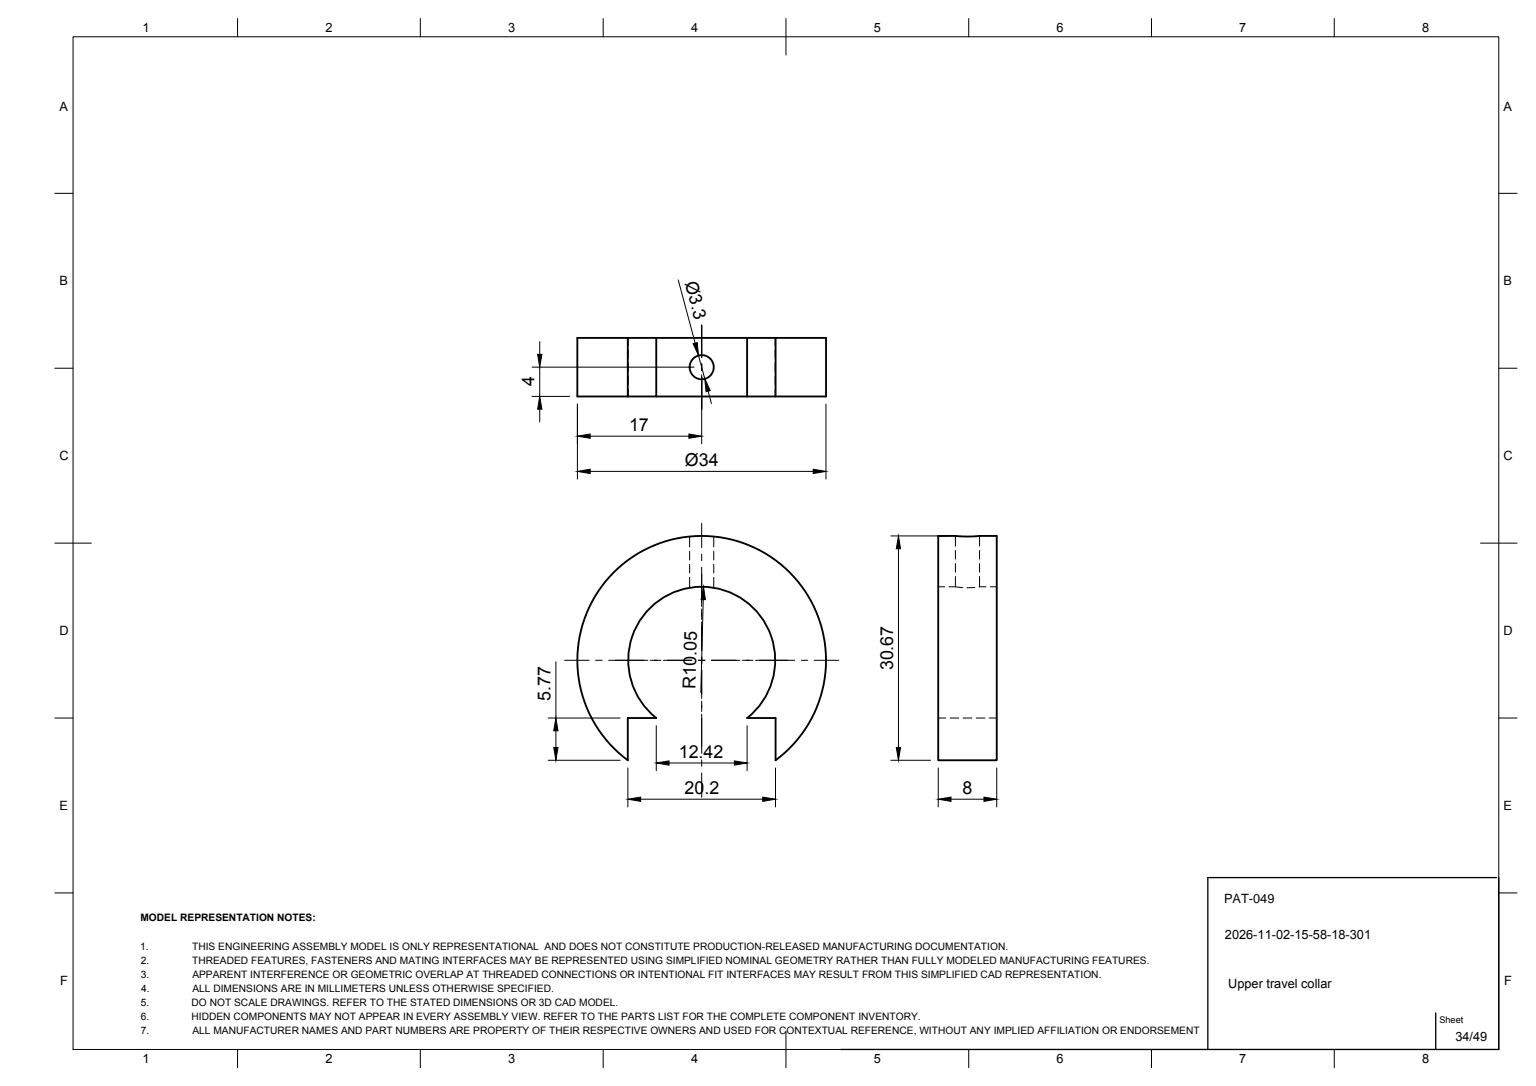
ISO-10303-21;
HEADER;
/* Generated by software containing ST-Developer
 * from STEP Tools, Inc. (www.steptools.com) 
 */

FILE_DESCRIPTION(
/* description */ ('Hand drill press frame (manual)'),
/* implementation_level */ '2;1');

FILE_NAME(
/* name */ 'Upper travel collar.step',
/* time_stamp */ '2026-10-28T03:25:28-07:00',
/* author */ (''),
/* organization */ (''),
/* preprocessor_version */ 'ST-DEVELOPER v20.2',
/* originating_system */ 'Autodesk Translation Framework v15.17.0.0',
/* authorisation */ '');

FILE_SCHEMA (('AUTOMOTIVE_DESIGN { 1 0 10303 214 3 1 1 }'));
ENDSEC;

DATA;
#10=MECHANICAL_DESIGN_GEOMETRIC_PRESENTATION_REPRESENTATION('',(#653),#33299);
#525=B_SPLINE_CURVE_WITH_KNOTS('',3,(#20892,#20893,#20894,#20895,#20896,
#20897,#20898,#20899,#20900,#20901),.UNSPECIFIED.,.F.,.F.,(4,2,2,2,4),(0.,
0.062275384959466,0.124550769918932,0.186824589898798,0.249098409878663),
 .UNSPECIFIED.);
#526=B_SPLINE_CURVE_WITH_KNOTS('',3,(#20902,#20903,#20904,#20905,#20906,
#20907,#20908,#20909,#20910,#20911,#20912,#20913,#20914,#20915,#20916,#20917,
#20918,#20919,#20920,#20921,#20922,#20923,#20924,#20925,#20926,#20927),
 .UNSPECIFIED.,.F.,.F.,(4,2,2,2,2,2,2,2,2,2,2,2,4),(0.249098409878663,0.311372229858529,
0.373646049838394,0.43592143479786,0.498196819757326,0.560472204716792,
0.622747589676259,0.685021409656124,0.74729522963599,0.809569049615855,
0.871842869595721,0.934118254555187,0.996393639514653),.UNSPECIFIED.);
#527=B_SPLINE_CURVE_WITH_KNOTS('',3,(#20931,#20932,#20933,#20934,#20935,
#20936,#20937,#20938,#20939,#20940,#20941,#20942,#20943,#20944,#20945,#20946,
#20947,#20948,#20949,#20950,#20951,#20952,#20953,#20954,#20955,#20956),
 .UNSPECIFIED.,.F.,.F.,(4,2,2,2,2,2,2,2,2,2,2,2,4),(0.,0.0621954302022363,
0.124390860404473,0.186586102839084,0.248781345273696,0.310976587708308,
0.37317183014292,0.435367260345156,0.497562690547392,0.559758120749629,
0.621953550951865,0.684148793386477,0.746344035821089),.UNSPECIFIED.);
#528=B_SPLINE_CURVE_WITH_KNOTS('',3,(#20957,#20958,#20959,#20960,#20961,
#20962,#20963,#20964,#20965,#20966),.UNSPECIFIED.,.F.,.F.,(4,2,2,2,4),(0.746344035821089,
0.8085392782557,0.870734520690312,0.932929950892549,0.995125381094785),
 .UNSPECIFIED.);
#556=SHAPE_REPRESENTATION_RELATIONSHIP('SRR','None',#33517,#601);
#601=ADVANCED_BREP_SHAPE_REPRESENTATION('',(#704),#33279);
#653=STYLED_ITEM('',(#33800),#704);
#704=MANIFOLD_SOLID_BREP('Body1',#12672);
#852=FACE_BOUND('',#2635,.T.);
#853=FACE_BOUND('',#2637,.T.);
#1223=PLANE('',#13969);
#1224=PLANE('',#13970);
#1225=PLANE('',#13971);
#1226=PLANE('',#13972);
#1227=PLANE('',#13973);
#1228=PLANE('',#13980);
#1807=FACE_OUTER_BOUND('',#2628,.T.);
#1808=FACE_OUTER_BOUND('',#2629,.T.);
#1809=FACE_OUTER_BOUND('',#2630,.T.);
#1810=FACE_OUTER_BOUND('',#2631,.T.);
#1811=FACE_OUTER_BOUND('',#2632,.T.);
#1812=FACE_OUTER_BOUND('',#2633,.T.);
#1813=FACE_OUTER_BOUND('',#2634,.T.);
#1814=FACE_OUTER_BOUND('',#2636,.T.);
#1815=FACE_OUTER_BOUND('',#2638,.T.);
#2628=EDGE_LOOP('',(#10769,#10770,#10771,#10772,#10773,#10774));
#2629=EDGE_LOOP('',(#10775,#10776,#10777,#10778));
#2630=EDGE_LOOP('',(#10779,#10780,#10781,#10782));
#2631=EDGE_LOOP('',(#10783,#10784,#10785,#10786));
#2632=EDGE_LOOP('',(#10787,#10788,#10789,#10790));
#2633=EDGE_LOOP('',(#10791,#10792,#10793,#10794,#10795,#10796));
#2634=EDGE_LOOP('',(#10797,#10798,#10799,#10800));
#2635=EDGE_LOOP('',(#10801,#10802));
#2636=EDGE_LOOP('',(#10803,#10804,#10805,#10806));
#2637=EDGE_LOOP('',(#10807,#10808));
#2638=EDGE_LOOP('',(#10809,#10810,#10811,#10812,#10813,#10814));
#3749=LINE('',#20929,#4914);
#3750=LINE('',#20970,#4915);
#3751=LINE('',#20972,#4916);
#3752=LINE('',#20974,#4917);
#3753=LINE('',#20975,#4918);
#3754=LINE('',#20979,#4919);
#3755=LINE('',#20981,#4920);
#3756=LINE('',#20983,#4921);
#3757=LINE('',#20984,#4922);
#3758=LINE('',#20987,#4923);
#3759=LINE('',#20989,#4924);
#3760=LINE('',#20990,#4925);
#3761=LINE('',#20993,#4926);
#3762=LINE('',#20995,#4927);
#3763=LINE('',#20996,#4928);
#4914=VECTOR('',#16794,0.164999999999999);
#4915=VECTOR('',#16797,1.);
#4916=VECTOR('',#16798,1.);
#4917=VECTOR('',#16799,1.);
#4918=VECTOR('',#16800,1.);
#4919=VECTOR('',#16803,1.);
#4920=VECTOR('',#16804,1.);
#4921=VECTOR('',#16805,1.);
#4922=VECTOR('',#16806,1.);
#4923=VECTOR('',#16809,1.);
#4924=VECTOR('',#16810,1.);
#4925=VECTOR('',#16811,1.);
#4926=VECTOR('',#16814,1.);
#4927=VECTOR('',#16815,1.);
#4928=VECTOR('',#16816,1.);
#5489=CIRCLE('',#13974,1.005);
#5490=CIRCLE('',#13975,1.7);
#5491=CIRCLE('',#13977,1.7);
#5492=CIRCLE('',#13979,1.005);
#6403=VERTEX_POINT('',#20890);
#6404=VERTEX_POINT('',#20891);
#6405=VERTEX_POINT('',#20928);
#6406=VERTEX_POINT('',#20930);
#6407=VERTEX_POINT('',#20968);
#6408=VERTEX_POINT('',#20969);
#6409=VERTEX_POINT('',#20971);
#6410=VERTEX_POINT('',#20973);
#6411=VERTEX_POINT('',#20977);
#6412=VERTEX_POINT('',#20978);
#6413=VERTEX_POINT('',#20980);
#6414=VERTEX_POINT('',#20982);
#6415=VERTEX_POINT('',#20986);
#6416=VERTEX_POINT('',#20988);
#6417=VERTEX_POINT('',#20992);
#6418=VERTEX_POINT('',#20994);
#7913=EDGE_CURVE('',#6403,#6404,#525,.T.);
#7914=EDGE_CURVE('',#6404,#6403,#526,.T.);
#7915=EDGE_CURVE('',#6404,#6405,#3749,.T.);
#7916=EDGE_CURVE('',#6406,#6405,#527,.T.);
#7917=EDGE_CURVE('',#6405,#6406,#528,.T.);
#7918=EDGE_CURVE('',#6407,#6408,#3750,.T.);
#7919=EDGE_CURVE('',#6407,#6409,#3751,.T.);
#7920=EDGE_CURVE('',#6410,#6409,#3752,.T.);
#7921=EDGE_CURVE('',#6408,#6410,#3753,.T.);
#7922=EDGE_CURVE('',#6411,#6412,#3754,.T.);
#7923=EDGE_CURVE('',#6411,#6413,#3755,.T.);
#7924=EDGE_CURVE('',#6414,#6413,#3756,.T.);
#7925=EDGE_CURVE('',#6412,#6414,#3757,.T.);
#7926=EDGE_CURVE('',#6415,#6407,#3758,.T.);
#7927=EDGE_CURVE('',#6416,#6415,#3759,.T.);
#7928=EDGE_CURVE('',#6409,#6416,#3760,.T.);
#7929=EDGE_CURVE('',#6417,#6411,#3761,.T.);
#7930=EDGE_CURVE('',#6418,#6417,#3762,.T.);
#7931=EDGE_CURVE('',#6413,#6418,#3763,.T.);
#7932=EDGE_CURVE('',#6416,#6414,#5489,.T.);
#7933=EDGE_CURVE('',#6418,#6410,#5490,.T.);
#7934=EDGE_CURVE('',#6417,#6408,#5491,.T.);
#7935=EDGE_CURVE('',#6415,#6412,#5492,.T.);
#10769=ORIENTED_EDGE('',*,*,#7913,.F.);
#10770=ORIENTED_EDGE('',*,*,#7914,.F.);
#10771=ORIENTED_EDGE('',*,*,#7915,.T.);
#10772=ORIENTED_EDGE('',*,*,#7916,.F.);
#10773=ORIENTED_EDGE('',*,*,#7917,.F.);
#10774=ORIENTED_EDGE('',*,*,#7915,.F.);
#10775=ORIENTED_EDGE('',*,*,#7918,.F.);
#10776=ORIENTED_EDGE('',*,*,#7919,.T.);
#10777=ORIENTED_EDGE('',*,*,#7920,.F.);
#10778=ORIENTED_EDGE('',*,*,#7921,.F.);
#10779=ORIENTED_EDGE('',*,*,#7922,.F.);
#10780=ORIENTED_EDGE('',*,*,#7923,.T.);
#10781=ORIENTED_EDGE('',*,*,#7924,.F.);
#10782=ORIENTED_EDGE('',*,*,#7925,.F.);
#10783=ORIENTED_EDGE('',*,*,#7926,.F.);
#10784=ORIENTED_EDGE('',*,*,#7927,.F.);
#10785=ORIENTED_EDGE('',*,*,#7928,.F.);
#10786=ORIENTED_EDGE('',*,*,#7919,.F.);
#10787=ORIENTED_EDGE('',*,*,#7929,.F.);
#10788=ORIENTED_EDGE('',*,*,#7930,.F.);
#10789=ORIENTED_EDGE('',*,*,#7931,.F.);
#10790=ORIENTED_EDGE('',*,*,#7923,.F.);
#10791=ORIENTED_EDGE('',*,*,#7920,.T.);
#10792=ORIENTED_EDGE('',*,*,#7928,.T.);
#10793=ORIENTED_EDGE('',*,*,#7932,.T.);
#10794=ORIENTED_EDGE('',*,*,#7924,.T.);
#10795=ORIENTED_EDGE('',*,*,#7931,.T.);
#10796=ORIENTED_EDGE('',*,*,#7933,.T.);
#10797=ORIENTED_EDGE('',*,*,#7921,.T.);
#10798=ORIENTED_EDGE('',*,*,#7933,.F.);
#10799=ORIENTED_EDGE('',*,*,#7930,.T.);
#10800=ORIENTED_EDGE('',*,*,#7934,.T.);
#10801=ORIENTED_EDGE('',*,*,#7916,.T.);
#10802=ORIENTED_EDGE('',*,*,#7917,.T.);
#10803=ORIENTED_EDGE('',*,*,#7927,.T.);
#10804=ORIENTED_EDGE('',*,*,#7935,.T.);
#10805=ORIENTED_EDGE('',*,*,#7925,.T.);
#10806=ORIENTED_EDGE('',*,*,#7932,.F.);
#10807=ORIENTED_EDGE('',*,*,#7913,.T.);
#10808=ORIENTED_EDGE('',*,*,#7914,.T.);
#10809=ORIENTED_EDGE('',*,*,#7918,.T.);
#10810=ORIENTED_EDGE('',*,*,#7934,.F.);
#10811=ORIENTED_EDGE('',*,*,#7929,.T.);
#10812=ORIENTED_EDGE('',*,*,#7922,.T.);
#10813=ORIENTED_EDGE('',*,*,#7935,.F.);
#10814=ORIENTED_EDGE('',*,*,#7926,.T.);
#11893=CYLINDRICAL_SURFACE('',#13968,0.164999999999999);
#11894=CYLINDRICAL_SURFACE('',#13976,1.7);
#11895=CYLINDRICAL_SURFACE('',#13978,1.005);
#12416=ADVANCED_FACE('',(#1807),#11893,.F.);
#12417=ADVANCED_FACE('',(#1808),#1223,.F.);
#12418=ADVANCED_FACE('',(#1809),#1224,.F.);
#12419=ADVANCED_FACE('',(#1810),#1225,.F.);
#12420=ADVANCED_FACE('',(#1811),#1226,.F.);
#12421=ADVANCED_FACE('',(#1812),#1227,.T.);
#12422=ADVANCED_FACE('',(#1813,#852),#11894,.T.);
#12423=ADVANCED_FACE('',(#1814,#853),#11895,.F.);
#12424=ADVANCED_FACE('',(#1815),#1228,.F.);
#12672=CLOSED_SHELL('',(#12416,#12417,#12418,#12419,#12420,#12421,#12422,
#12423,#12424));
#13967=AXIS2_PLACEMENT_3D('',#20888,#16790,#16791);
#13968=AXIS2_PLACEMENT_3D('',#20889,#16792,#16793);
#13969=AXIS2_PLACEMENT_3D('',#20967,#16795,#16796);
#13970=AXIS2_PLACEMENT_3D('',#20976,#16801,#16802);
#13971=AXIS2_PLACEMENT_3D('',#20985,#16807,#16808);
#13972=AXIS2_PLACEMENT_3D('',#20991,#16812,#16813);
#13973=AXIS2_PLACEMENT_3D('',#20997,#16817,#16818);
#13974=AXIS2_PLACEMENT_3D('',#20998,#16819,#16820);
#13975=AXIS2_PLACEMENT_3D('',#20999,#16821,#16822);
#13976=AXIS2_PLACEMENT_3D('',#21000,#16823,#16824);
#13977=AXIS2_PLACEMENT_3D('',#21001,#16825,#16826);
#13978=AXIS2_PLACEMENT_3D('',#21002,#16827,#16828);
#13979=AXIS2_PLACEMENT_3D('',#21003,#16829,#16830);
#13980=AXIS2_PLACEMENT_3D('',#21004,#16831,#16832);
#16790=DIRECTION('axis',(0.,0.,1.));
#16791=DIRECTION('refdir',(1.,0.,0.));
#16792=DIRECTION('center_axis',(1.,0.,0.));
#16793=DIRECTION('ref_axis',(0.,0.,-1.));
#16794=DIRECTION('',(1.,0.,0.));
#16795=DIRECTION('center_axis',(0.,1.,0.));
#16796=DIRECTION('ref_axis',(-1.,0.,0.));
#16797=DIRECTION('',(-1.,0.,0.));
#16798=DIRECTION('',(0.,0.,1.));
#16799=DIRECTION('',(1.,0.,0.));
#16800=DIRECTION('',(0.,0.,1.));
#16801=DIRECTION('center_axis',(1.,0.,0.));
#16802=DIRECTION('ref_axis',(0.,1.,0.));
#16803=DIRECTION('',(0.,1.,0.));
#16804=DIRECTION('',(0.,0.,1.));
#16805=DIRECTION('',(0.,-1.,0.));
#16806=DIRECTION('',(0.,0.,1.));
#16807=DIRECTION('center_axis',(1.,0.,0.));
#16808=DIRECTION('ref_axis',(0.,1.,0.));
#16809=DIRECTION('',(0.,1.,0.));
#16810=DIRECTION('',(0.,0.,-1.));
#16811=DIRECTION('',(0.,-1.,0.));
#16812=DIRECTION('center_axis',(0.,-1.,0.));
#16813=DIRECTION('ref_axis',(1.,0.,0.));
#16814=DIRECTION('',(1.,0.,0.));
#16815=DIRECTION('',(0.,0.,-1.));
#16816=DIRECTION('',(-1.,0.,0.));
#16817=DIRECTION('center_axis',(0.,0.,1.));
#16818=DIRECTION('ref_axis',(1.,0.,0.));
#16819=DIRECTION('center_axis',(0.,0.,-1.));
#16820=DIRECTION('ref_axis',(1.,0.,0.));
#16821=DIRECTION('center_axis',(0.,0.,1.));
#16822=DIRECTION('ref_axis',(1.,0.,0.));
#16823=DIRECTION('center_axis',(0.,0.,1.));
#16824=DIRECTION('ref_axis',(1.,0.,0.));
#16825=DIRECTION('center_axis',(0.,0.,1.));
#16826=DIRECTION('ref_axis',(1.,0.,0.));
#16827=DIRECTION('center_axis',(0.,0.,1.));
#16828=DIRECTION('ref_axis',(1.,0.,0.));
#16829=DIRECTION('center_axis',(0.,0.,-1.));
#16830=DIRECTION('ref_axis',(1.,0.,0.));
#16831=DIRECTION('center_axis',(0.,0.,1.));
#16832=DIRECTION('ref_axis',(1.,0.,0.));
#20888=CARTESIAN_POINT('',(0.,0.,0.));
#20889=CARTESIAN_POINT('Origin',(1.99,0.,30.));
#20890=CARTESIAN_POINT('',(1.9913626985115,0.164999999999999,30.));
#20891=CARTESIAN_POINT('',(2.005,-8.29617220839915E-17,30.165));
#20892=CARTESIAN_POINT('Ctrl Pts',(1.9913626985115,0.164999999999999,30.));
#20893=CARTESIAN_POINT('Ctrl Pts',(1.9913626985115,0.164999999999999,30.0207584616532));
#20894=CARTESIAN_POINT('Ctrl Pts',(1.99208213234536,0.160843707720236,30.0428743626922));
#20895=CARTESIAN_POINT('Ctrl Pts',(1.99466757507705,0.143993298000808,30.0835155100945));
#20896=CARTESIAN_POINT('Ctrl Pts',(1.9964948147884,0.131301190829395,30.1020440469622));
#20897=CARTESIAN_POINT('Ctrl Pts',(1.99991441892026,0.102044414577984,30.1313008232136));
#20898=CARTESIAN_POINT('Ctrl Pts',(2.00173085232892,0.0835157197655822,
30.1439932187437));
#20899=CARTESIAN_POINT('Ctrl Pts',(2.00429148829838,0.0428740302308141,
30.1608438378879));
#20900=CARTESIAN_POINT('Ctrl Pts',(2.005,0.0207579399932888,30.165));
#20901=CARTESIAN_POINT('Ctrl Pts',(2.005,2.35922392732846E-16,30.165));
#20902=CARTESIAN_POINT('Ctrl Pts',(2.005,-1.52655665885959E-16,30.165));
#20903=CARTESIAN_POINT('Ctrl Pts',(2.005,-0.0207579399932887,30.165));
#20904=CARTESIAN_POINT('Ctrl Pts',(2.00429148829838,-0.0428740302308141,
30.1608438378879));
#20905=CARTESIAN_POINT('Ctrl Pts',(2.00173085232892,-0.0835157197655809,
30.1439932187437));
#20906=CARTESIAN_POINT('Ctrl Pts',(1.99991441892026,-0.102044414577984,
30.1313008232136));
#20907=CARTESIAN_POINT('Ctrl Pts',(1.9964948147884,-0.131301190829395,30.1020440469622));
#20908=CARTESIAN_POINT('Ctrl Pts',(1.99466757507705,-0.143993298000808,
30.0835155100945));
#20909=CARTESIAN_POINT('Ctrl Pts',(1.99208213234536,-0.160843707720236,
30.0428743626922));
#20910=CARTESIAN_POINT('Ctrl Pts',(1.9913626985115,-0.164999999999999,30.0207584616532));
#20911=CARTESIAN_POINT('Ctrl Pts',(1.9913626985115,-0.164999999999999,29.9792415383468));
#20912=CARTESIAN_POINT('Ctrl Pts',(1.99208213234536,-0.160843707720236,
29.9571256373078));
#20913=CARTESIAN_POINT('Ctrl Pts',(1.99466757507705,-0.143993298000808,
29.9164844899055));
#20914=CARTESIAN_POINT('Ctrl Pts',(1.9964948147884,-0.131301190829395,29.8979559530378));
#20915=CARTESIAN_POINT('Ctrl Pts',(1.99991441892026,-0.102044414577984,
29.8686991767864));
#20916=CARTESIAN_POINT('Ctrl Pts',(2.00173085232892,-0.0835157197655809,
29.8560067812563));
#20917=CARTESIAN_POINT('Ctrl Pts',(2.00429148829838,-0.0428740302308141,
29.8391561621121));
#20918=CARTESIAN_POINT('Ctrl Pts',(2.005,-0.0207579399932886,29.835));
#20919=CARTESIAN_POINT('Ctrl Pts',(2.005,0.0207579399932885,29.835));
#20920=CARTESIAN_POINT('Ctrl Pts',(2.00429148829838,0.042874030230814,29.8391561621121));
#20921=CARTESIAN_POINT('Ctrl Pts',(2.00173085232892,0.0835157197655809,
29.8560067812563));
#20922=CARTESIAN_POINT('Ctrl Pts',(1.99991441892026,0.102044414577984,29.8686991767864));
#20923=CARTESIAN_POINT('Ctrl Pts',(1.9964948147884,0.131301190829395,29.8979559530378));
#20924=CARTESIAN_POINT('Ctrl Pts',(1.99466757507705,0.143993298000808,29.9164844899055));
#20925=CARTESIAN_POINT('Ctrl Pts',(1.99208213234536,0.160843707720236,29.9571256373078));
#20926=CARTESIAN_POINT('Ctrl Pts',(1.9913626985115,0.164999999999999,29.9792415383468));
#20927=CARTESIAN_POINT('Ctrl Pts',(1.9913626985115,0.164999999999999,30.));
#20928=CARTESIAN_POINT('',(2.7,-2.02066721859312E-17,30.165));
#20929=CARTESIAN_POINT('',(1.99,-2.02066721859312E-17,30.165));
#20930=CARTESIAN_POINT('',(2.69197369955919,0.164999999999999,30.));
#20931=CARTESIAN_POINT('Ctrl Pts',(2.69197369955919,0.164999999999999,30.));
#20932=CARTESIAN_POINT('Ctrl Pts',(2.69197369955919,0.164999999999999,29.9792681899326));
#20933=CARTESIAN_POINT('Ctrl Pts',(2.69239400387291,0.160854068850877,29.9571634685398));
#20934=CARTESIAN_POINT('Ctrl Pts',(2.69391035162893,0.14401116680132,29.9165147673388));
#20935=CARTESIAN_POINT('Ctrl Pts',(2.69498430847444,0.13131490896209,29.8979696711705));
#20936=CARTESIAN_POINT('Ctrl Pts',(2.69699888419766,0.102030373034454,29.8686851352429));
#20937=CARTESIAN_POINT('Ctrl Pts',(2.69807062966546,0.0834852574625918,
29.8559888429375));
#20938=CARTESIAN_POINT('Ctrl Pts',(2.69958191522061,0.0428364913743715,
29.8391459150772));
#20939=CARTESIAN_POINT('Ctrl Pts',(2.7,0.0207317474782039,29.835));
#20940=CARTESIAN_POINT('Ctrl Pts',(2.7,-0.0207317474782039,29.835));
#20941=CARTESIAN_POINT('Ctrl Pts',(2.69958191522061,-0.0428364913743715,
29.8391459150772));
#20942=CARTESIAN_POINT('Ctrl Pts',(2.69807062966546,-0.0834852574625918,
29.8559888429375));
#20943=CARTESIAN_POINT('Ctrl Pts',(2.69699888419766,-0.102030373034454,
29.8686851352429));
#20944=CARTESIAN_POINT('Ctrl Pts',(2.69498430847444,-0.13131490896209,29.8979696711705));
#20945=CARTESIAN_POINT('Ctrl Pts',(2.69391035162893,-0.14401116680132,29.9165147673388));
#20946=CARTESIAN_POINT('Ctrl Pts',(2.69239400387291,-0.160854068850877,
29.9571634685398));
#20947=CARTESIAN_POINT('Ctrl Pts',(2.69197369955919,-0.164999999999999,
29.9792681899326));
#20948=CARTESIAN_POINT('Ctrl Pts',(2.69197369955919,-0.164999999999999,
30.0207318100674));
#20949=CARTESIAN_POINT('Ctrl Pts',(2.69239400387291,-0.160854068850877,
30.0428365314602));
#20950=CARTESIAN_POINT('Ctrl Pts',(2.69391035162893,-0.14401116680132,30.0834852326612));
#20951=CARTESIAN_POINT('Ctrl Pts',(2.69498430847444,-0.13131490896209,30.1020303288295));
#20952=CARTESIAN_POINT('Ctrl Pts',(2.69699888419766,-0.102030373034454,
30.1313148647571));
#20953=CARTESIAN_POINT('Ctrl Pts',(2.69807062966546,-0.0834852574625918,
30.1440111570625));
#20954=CARTESIAN_POINT('Ctrl Pts',(2.69958191522061,-0.0428364913743716,
30.1608540849228));
#20955=CARTESIAN_POINT('Ctrl Pts',(2.7,-0.0207317474782039,30.165));
#20956=CARTESIAN_POINT('Ctrl Pts',(2.7,6.24500451351651E-17,30.165));
#20957=CARTESIAN_POINT('Ctrl Pts',(2.7,-1.11022302462516E-16,30.165));
#20958=CARTESIAN_POINT('Ctrl Pts',(2.7,0.0207317474782038,30.165));
#20959=CARTESIAN_POINT('Ctrl Pts',(2.69958191522061,0.0428364913743715,
30.1608540849228));
#20960=CARTESIAN_POINT('Ctrl Pts',(2.69807062966546,0.0834852574625918,
30.1440111570625));
#20961=CARTESIAN_POINT('Ctrl Pts',(2.69699888419766,0.102030373034454,30.1313148647571));
#20962=CARTESIAN_POINT('Ctrl Pts',(2.69498430847444,0.13131490896209,30.1020303288295));
#20963=CARTESIAN_POINT('Ctrl Pts',(2.69391035162893,0.14401116680132,30.0834852326612));
#20964=CARTESIAN_POINT('Ctrl Pts',(2.69239400387291,0.160854068850877,30.0428365314602));
#20965=CARTESIAN_POINT('Ctrl Pts',(2.69197369955919,0.164999999999999,30.0207318100674));
#20966=CARTESIAN_POINT('Ctrl Pts',(2.69197369955919,0.164999999999999,30.));
#20967=CARTESIAN_POINT('Origin',(0.21,1.01,29.5));
#20968=CARTESIAN_POINT('',(0.21,1.01,29.6));
#20969=CARTESIAN_POINT('',(-0.367442869007697,1.01,29.6));
#20970=CARTESIAN_POINT('',(0.605,1.01,29.6));
#20971=CARTESIAN_POINT('',(0.21,1.01,30.4));
#20972=CARTESIAN_POINT('',(0.21,1.01,29.5));
#20973=CARTESIAN_POINT('',(-0.367442869007697,1.01,30.4));
#20974=CARTESIAN_POINT('',(0.605,1.01,30.4));
#20975=CARTESIAN_POINT('',(-0.367442869007697,1.01,29.6));
#20976=CARTESIAN_POINT('Origin',(0.21,-1.01,29.5));
#20977=CARTESIAN_POINT('',(0.21,-1.01,29.6));
#20978=CARTESIAN_POINT('',(0.21,-0.621228621362538,29.6));
#20979=CARTESIAN_POINT('',(0.21,-0.505,29.6));
#20980=CARTESIAN_POINT('',(0.21,-1.01,30.4));
#20981=CARTESIAN_POINT('',(0.21,-1.01,29.5));
#20982=CARTESIAN_POINT('',(0.21,-0.621228621362538,30.4));
#20983=CARTESIAN_POINT('',(0.21,-0.505,30.4));
#20984=CARTESIAN_POINT('',(0.21,-0.621228621362538,29.6));
#20985=CARTESIAN_POINT('Origin',(0.21,-1.01,29.5));
#20986=CARTESIAN_POINT('',(0.21,0.621228621362538,29.6));
#20987=CARTESIAN_POINT('',(0.21,-0.505,29.6));
#20988=CARTESIAN_POINT('',(0.21,0.621228621362538,30.4));
#20989=CARTESIAN_POINT('',(0.21,0.621228621362538,29.6));
#20990=CARTESIAN_POINT('',(0.21,-0.505,30.4));
#20991=CARTESIAN_POINT('Origin',(-0.8,-1.01,29.5));
#20992=CARTESIAN_POINT('',(-0.367442869007697,-1.01,29.6));
#20993=CARTESIAN_POINT('',(0.1,-1.01,29.6));
#20994=CARTESIAN_POINT('',(-0.367442869007697,-1.01,30.4));
#20995=CARTESIAN_POINT('',(-0.367442869007697,-1.01,29.6));
#20996=CARTESIAN_POINT('',(0.1,-1.01,30.4));
#20997=CARTESIAN_POINT('Origin',(1.,0.,30.4));
#20998=CARTESIAN_POINT('Origin',(1.,0.,30.4));
#20999=CARTESIAN_POINT('Origin',(1.,0.,30.4));
#21000=CARTESIAN_POINT('Origin',(1.,0.,29.6));
#21001=CARTESIAN_POINT('Origin',(1.,0.,29.6));
#21002=CARTESIAN_POINT('Origin',(1.,0.,29.6));
#21003=CARTESIAN_POINT('Origin',(1.,0.,29.6));
#21004=CARTESIAN_POINT('Origin',(1.,0.,29.6));
#33227=UNCERTAINTY_MEASURE_WITH_UNIT(LENGTH_MEASURE(0.001),#33300,
'DISTANCE_ACCURACY_VALUE',
'Maximum model space distance between geometric entities at asserted c
onnectivities');
#33247=UNCERTAINTY_MEASURE_WITH_UNIT(LENGTH_MEASURE(0.001),#33300,
'DISTANCE_ACCURACY_VALUE',
'Maximum model space distance between geometric entities at asserted c
onnectivities');
#33279=(
GEOMETRIC_REPRESENTATION_CONTEXT(3)
GLOBAL_UNCERTAINTY_ASSIGNED_CONTEXT((#33227))
GLOBAL_UNIT_ASSIGNED_CONTEXT((#33300,#33302,#33303))
REPRESENTATION_CONTEXT('','3D')
);
#33299=(
GEOMETRIC_REPRESENTATION_CONTEXT(3)
GLOBAL_UNCERTAINTY_ASSIGNED_CONTEXT((#33247))
GLOBAL_UNIT_ASSIGNED_CONTEXT((#33300,#33302,#33303))
REPRESENTATION_CONTEXT('','3D')
);
#33300=(
LENGTH_UNIT()
NAMED_UNIT(*)
SI_UNIT(.CENTI.,.METRE.)
);
#33302=(
NAMED_UNIT(*)
PLANE_ANGLE_UNIT()
SI_UNIT($,.RADIAN.)
);
#33303=(
NAMED_UNIT(*)
SI_UNIT($,.STERADIAN.)
SOLID_ANGLE_UNIT()
);
#33335=SHAPE_DEFINITION_REPRESENTATION(#33391,#33517);
#33391=PRODUCT_DEFINITION_SHAPE('',$,#33569);
#33517=SHAPE_REPRESENTATION('',(#13967),#33279);
#33537=PRODUCT_DEFINITION_CONTEXT('part definition',#33692,'design');
#33569=PRODUCT_DEFINITION('Upper travel collar','Upper travel collar',#33620,
#33537);
#33620=PRODUCT_DEFINITION_FORMATION('',$,#33725);
#33692=APPLICATION_CONTEXT(
'Core Data for Automotive Mechanical Design Process');
#33693=PRODUCT_CONTEXT('part definition',#33692,'mechanical');
#33725=PRODUCT('Upper travel collar','Upper travel collar',
'Upper travel collar',(#33693));
#33794=COLOUR_RGB('Light Blue',0.38,0.62,0.78);
#33795=FILL_AREA_STYLE_COLOUR('',#33794);
#33796=FILL_AREA_STYLE('',(#33795));
#33797=SURFACE_STYLE_FILL_AREA(#33796);
#33798=SURFACE_SIDE_STYLE('',(#33797));
#33799=SURFACE_STYLE_USAGE(.BOTH.,#33798);
#33800=PRESENTATION_STYLE_ASSIGNMENT((#33799));
ENDSEC;
END-ISO-10303-21;
